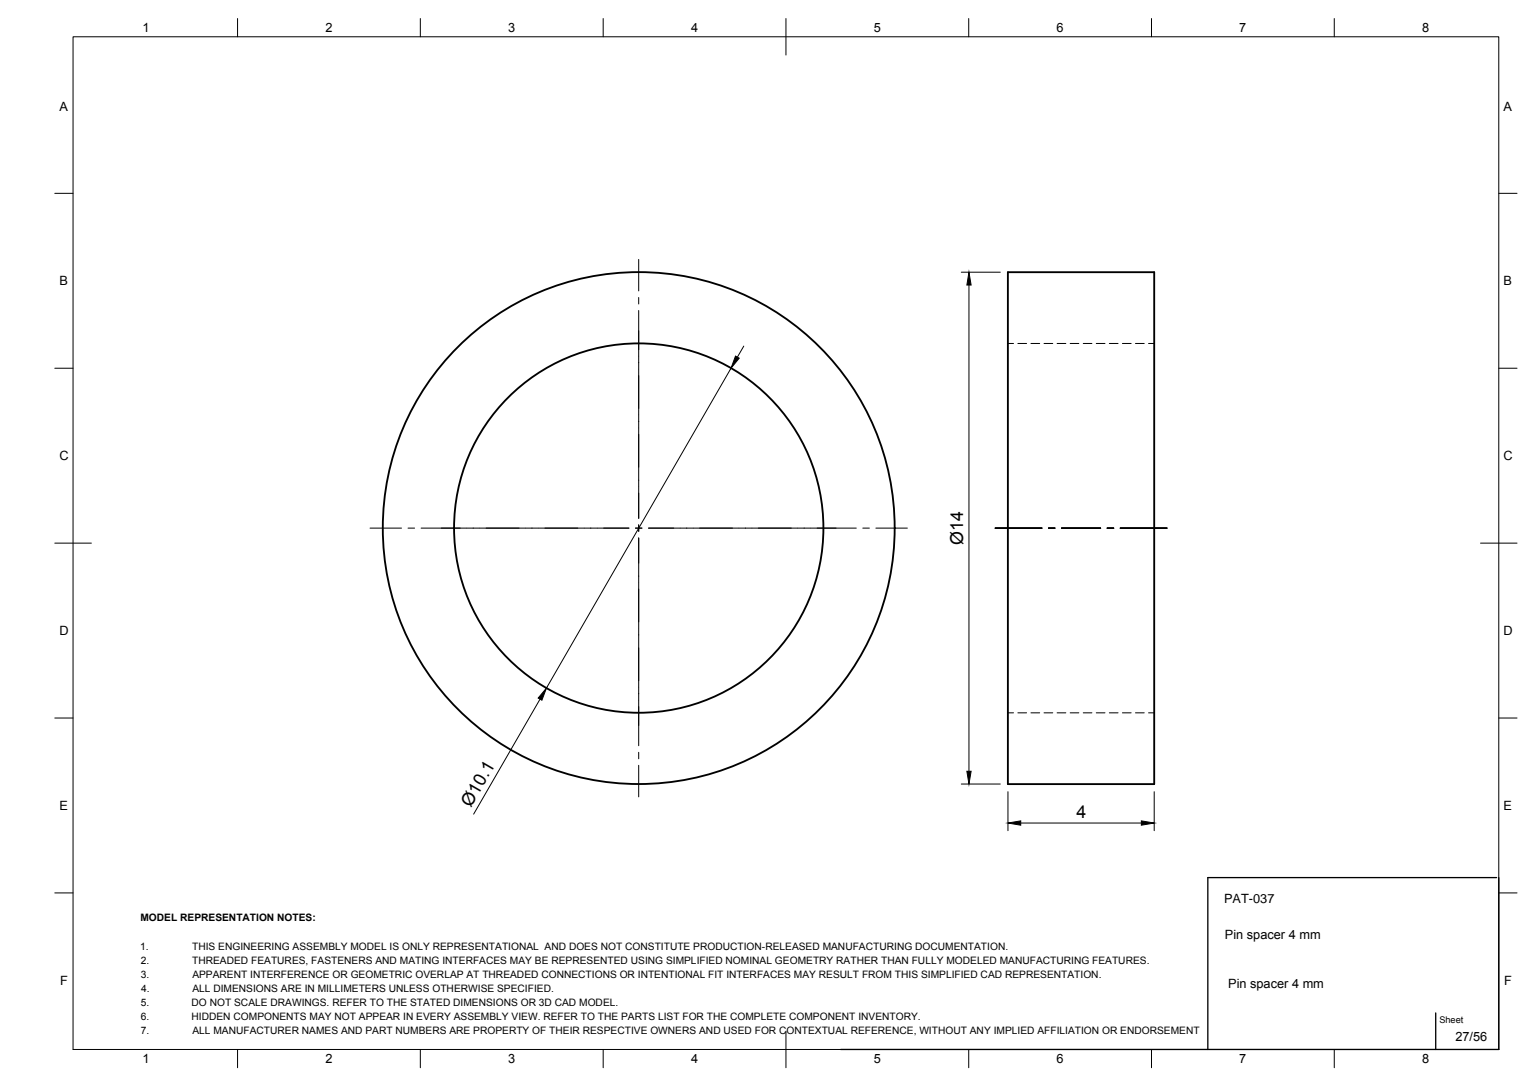
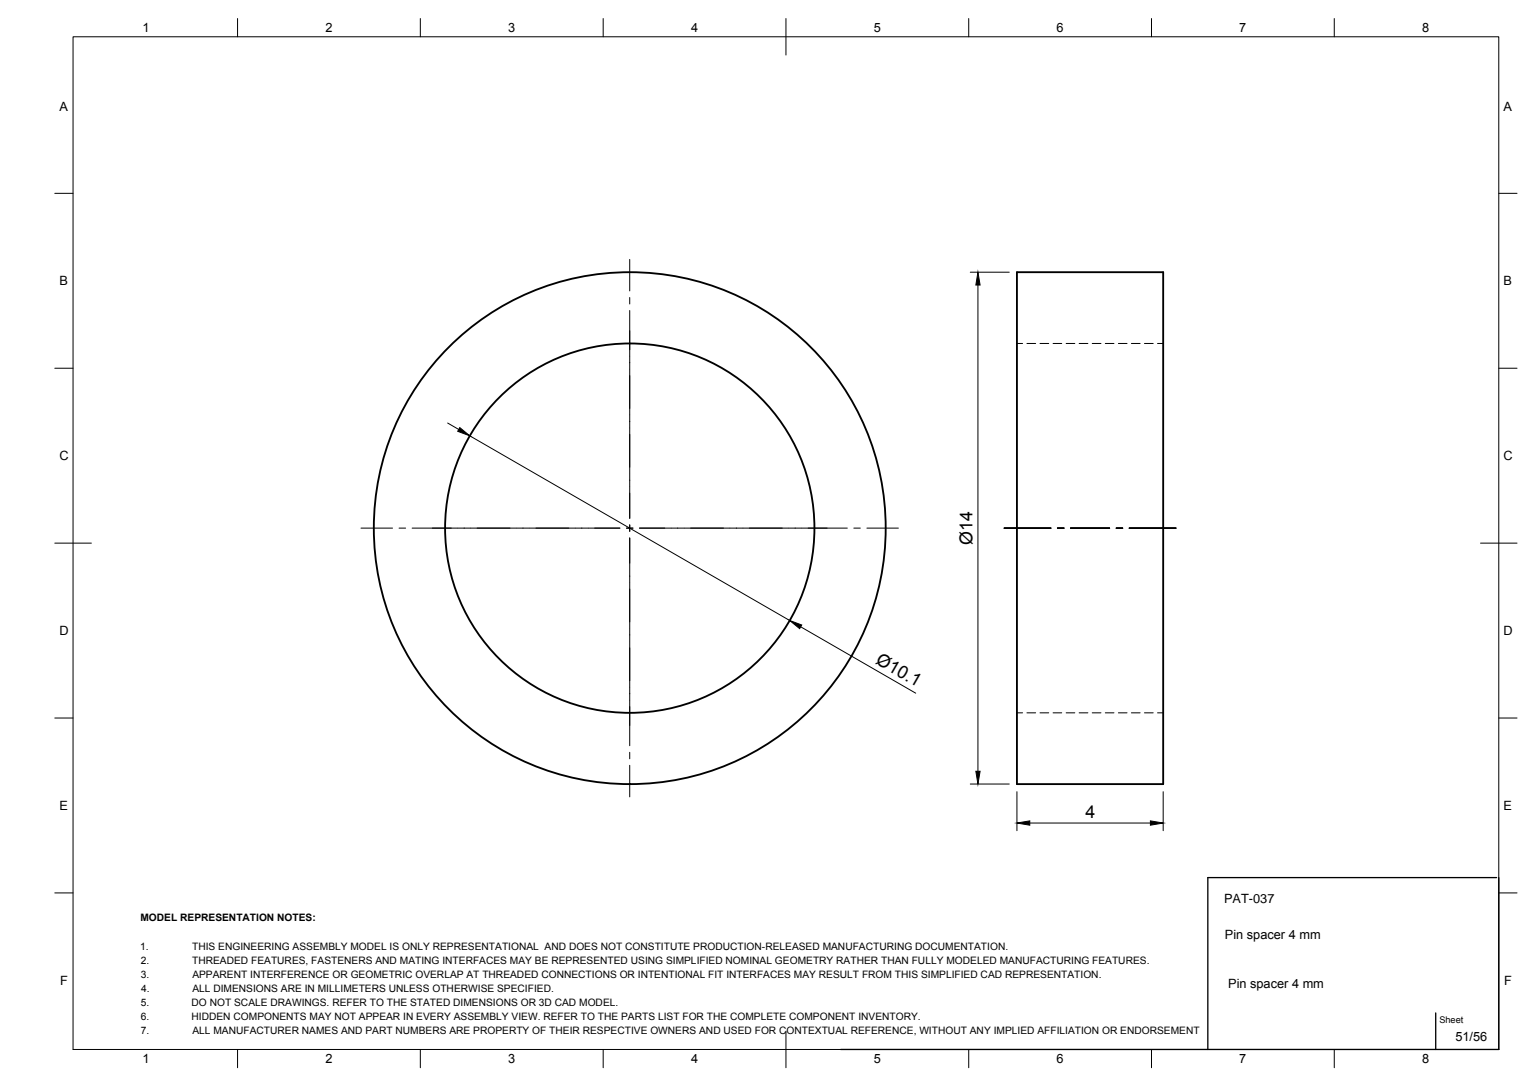
ISO-10303-21;
HEADER;
/* Generated by software containing ST-Developer
 * from STEP Tools, Inc. (www.steptools.com) 
 */

FILE_DESCRIPTION(
/* description */ ('Flywheel Crank-Slider'),
/* implementation_level */ '2;1');

FILE_NAME(
/* name */ 'Pin spacer 4 mm.step',
/* time_stamp */ '2026-10-28T03:23:13-07:00',
/* author */ (''),
/* organization */ (''),
/* preprocessor_version */ 'ST-DEVELOPER v20.2',
/* originating_system */ 'Autodesk Translation Framework v15.17.0.0',
/* authorisation */ '');

FILE_SCHEMA (('AUTOMOTIVE_DESIGN { 1 0 10303 214 3 1 1 }'));
ENDSEC;

DATA;
#10=MECHANICAL_DESIGN_GEOMETRIC_PRESENTATION_REPRESENTATION('',(#697),#17322);
#592=SHAPE_REPRESENTATION_RELATIONSHIP('SRR','None',#17590,#644);
#644=ADVANCED_BREP_SHAPE_REPRESENTATION('',(#754),#17294);
#697=STYLED_ITEM('',(#17931),#754);
#754=MANIFOLD_SOLID_BREP('Body1',#9079);
#926=FACE_BOUND('',#2327,.T.);
#927=FACE_BOUND('',#2329,.T.);
#1207=PLANE('',#10300);
#1208=PLANE('',#10301);
#1648=FACE_OUTER_BOUND('',#2324,.T.);
#1649=FACE_OUTER_BOUND('',#2325,.T.);
#1650=FACE_OUTER_BOUND('',#2326,.T.);
#1651=FACE_OUTER_BOUND('',#2328,.T.);
#2324=EDGE_LOOP('',(#7492,#7493,#7494,#7495));
#2325=EDGE_LOOP('',(#7496,#7497,#7498,#7499));
#2326=EDGE_LOOP('',(#7500));
#2327=EDGE_LOOP('',(#7501));
#2328=EDGE_LOOP('',(#7502));
#2329=EDGE_LOOP('',(#7503));
#3019=LINE('',#15818,#3630);
#3020=LINE('',#15824,#3631);
#3630=VECTOR('',#12455,0.505);
#3631=VECTOR('',#12462,0.7);
#4084=CIRCLE('',#10295,0.505);
#4085=CIRCLE('',#10296,0.505);
#4086=CIRCLE('',#10298,0.7);
#4087=CIRCLE('',#10299,0.7);
#4731=VERTEX_POINT('',#15815);
#4732=VERTEX_POINT('',#15817);
#4733=VERTEX_POINT('',#15821);
#4734=VERTEX_POINT('',#15823);
#5703=EDGE_CURVE('',#4731,#4731,#4084,.T.);
#5704=EDGE_CURVE('',#4731,#4732,#3019,.T.);
#5705=EDGE_CURVE('',#4732,#4732,#4085,.T.);
#5706=EDGE_CURVE('',#4733,#4733,#4086,.T.);
#5707=EDGE_CURVE('',#4733,#4734,#3020,.T.);
#5708=EDGE_CURVE('',#4734,#4734,#4087,.T.);
#7492=ORIENTED_EDGE('',*,*,#5703,.F.);
#7493=ORIENTED_EDGE('',*,*,#5704,.T.);
#7494=ORIENTED_EDGE('',*,*,#5705,.T.);
#7495=ORIENTED_EDGE('',*,*,#5704,.F.);
#7496=ORIENTED_EDGE('',*,*,#5706,.F.);
#7497=ORIENTED_EDGE('',*,*,#5707,.T.);
#7498=ORIENTED_EDGE('',*,*,#5708,.T.);
#7499=ORIENTED_EDGE('',*,*,#5707,.F.);
#7500=ORIENTED_EDGE('',*,*,#5706,.T.);
#7501=ORIENTED_EDGE('',*,*,#5703,.T.);
#7502=ORIENTED_EDGE('',*,*,#5708,.F.);
#7503=ORIENTED_EDGE('',*,*,#5705,.F.);
#8444=CYLINDRICAL_SURFACE('',#10294,0.505);
#8445=CYLINDRICAL_SURFACE('',#10297,0.7);
#8839=ADVANCED_FACE('',(#1648),#8444,.F.);
#8840=ADVANCED_FACE('',(#1649),#8445,.T.);
#8841=ADVANCED_FACE('',(#1650,#926),#1207,.T.);
#8842=ADVANCED_FACE('',(#1651,#927),#1208,.F.);
#9079=CLOSED_SHELL('',(#8839,#8840,#8841,#8842));
#10293=AXIS2_PLACEMENT_3D('',#15813,#12449,#12450);
#10294=AXIS2_PLACEMENT_3D('',#15814,#12451,#12452);
#10295=AXIS2_PLACEMENT_3D('',#15816,#12453,#12454);
#10296=AXIS2_PLACEMENT_3D('',#15819,#12456,#12457);
#10297=AXIS2_PLACEMENT_3D('',#15820,#12458,#12459);
#10298=AXIS2_PLACEMENT_3D('',#15822,#12460,#12461);
#10299=AXIS2_PLACEMENT_3D('',#15825,#12463,#12464);
#10300=AXIS2_PLACEMENT_3D('',#15826,#12465,#12466);
#10301=AXIS2_PLACEMENT_3D('',#15827,#12467,#12468);
#12449=DIRECTION('axis',(0.,0.,1.));
#12450=DIRECTION('refdir',(1.,0.,0.));
#12451=DIRECTION('center_axis',(0.,1.,0.));
#12452=DIRECTION('ref_axis',(1.,0.,0.));
#12453=DIRECTION('center_axis',(0.,-1.,0.));
#12454=DIRECTION('ref_axis',(1.,0.,0.));
#12455=DIRECTION('',(0.,-1.,0.));
#12456=DIRECTION('center_axis',(0.,-1.,0.));
#12457=DIRECTION('ref_axis',(1.,0.,0.));
#12458=DIRECTION('center_axis',(0.,1.,0.));
#12459=DIRECTION('ref_axis',(1.,0.,0.));
#12460=DIRECTION('center_axis',(0.,1.,0.));
#12461=DIRECTION('ref_axis',(1.,0.,0.));
#12462=DIRECTION('',(0.,-1.,0.));
#12463=DIRECTION('center_axis',(0.,1.,0.));
#12464=DIRECTION('ref_axis',(1.,0.,0.));
#12465=DIRECTION('center_axis',(0.,1.,0.));
#12466=DIRECTION('ref_axis',(1.,0.,0.));
#12467=DIRECTION('center_axis',(0.,1.,0.));
#12468=DIRECTION('ref_axis',(1.,0.,0.));
#15813=CARTESIAN_POINT('',(0.,0.,0.));
#15814=CARTESIAN_POINT('Origin',(2.,3.4,10.));
#15815=CARTESIAN_POINT('',(1.495,3.8,10.));
#15816=CARTESIAN_POINT('Origin',(2.,3.8,10.));
#15817=CARTESIAN_POINT('',(1.495,3.4,10.));
#15818=CARTESIAN_POINT('',(1.495,3.4,10.));
#15819=CARTESIAN_POINT('Origin',(2.,3.4,10.));
#15820=CARTESIAN_POINT('Origin',(2.,3.4,10.));
#15821=CARTESIAN_POINT('',(1.3,3.8,10.));
#15822=CARTESIAN_POINT('Origin',(2.,3.8,10.));
#15823=CARTESIAN_POINT('',(1.3,3.4,10.));
#15824=CARTESIAN_POINT('',(1.3,3.4,10.));
#15825=CARTESIAN_POINT('Origin',(2.,3.4,10.));
#15826=CARTESIAN_POINT('Origin',(2.,3.8,10.));
#15827=CARTESIAN_POINT('Origin',(2.,3.4,10.));
#17233=UNCERTAINTY_MEASURE_WITH_UNIT(LENGTH_MEASURE(0.001),#17323,
'DISTANCE_ACCURACY_VALUE',
'Maximum model space distance between geometric entities at asserted c
onnectivities');
#17261=UNCERTAINTY_MEASURE_WITH_UNIT(LENGTH_MEASURE(0.001),#17323,
'DISTANCE_ACCURACY_VALUE',
'Maximum model space distance between geometric entities at asserted c
onnectivities');
#17294=(
GEOMETRIC_REPRESENTATION_CONTEXT(3)
GLOBAL_UNCERTAINTY_ASSIGNED_CONTEXT((#17233))
GLOBAL_UNIT_ASSIGNED_CONTEXT((#17323,#17325,#17326))
REPRESENTATION_CONTEXT('','3D')
);
#17322=(
GEOMETRIC_REPRESENTATION_CONTEXT(3)
GLOBAL_UNCERTAINTY_ASSIGNED_CONTEXT((#17261))
GLOBAL_UNIT_ASSIGNED_CONTEXT((#17323,#17325,#17326))
REPRESENTATION_CONTEXT('','3D')
);
#17323=(
LENGTH_UNIT()
NAMED_UNIT(*)
SI_UNIT(.CENTI.,.METRE.)
);
#17325=(
NAMED_UNIT(*)
PLANE_ANGLE_UNIT()
SI_UNIT($,.RADIAN.)
);
#17326=(
NAMED_UNIT(*)
SI_UNIT($,.STERADIAN.)
SOLID_ANGLE_UNIT()
);
#17359=SHAPE_DEFINITION_REPRESENTATION(#17421,#17590);
#17421=PRODUCT_DEFINITION_SHAPE('',$,#17651);
#17590=SHAPE_REPRESENTATION('',(#10293),#17294);
#17618=PRODUCT_DEFINITION_CONTEXT('part definition',#17800,'design');
#17651=PRODUCT_DEFINITION('Pin spacer 4 mm','Pin spacer 4 mm',#17711,#17618);
#17711=PRODUCT_DEFINITION_FORMATION('',$,#17834);
#17800=APPLICATION_CONTEXT(
'Core Data for Automotive Mechanical Design Process');
#17801=PRODUCT_CONTEXT('part definition',#17800,'mechanical');
#17834=PRODUCT('Pin spacer 4 mm','Pin spacer 4 mm','Pin spacer 4 mm',(#17801));
#17925=COLOUR_RGB('Grey',0.48,0.52,0.57);
#17926=FILL_AREA_STYLE_COLOUR('',#17925);
#17927=FILL_AREA_STYLE('',(#17926));
#17928=SURFACE_STYLE_FILL_AREA(#17927);
#17929=SURFACE_SIDE_STYLE('',(#17928));
#17930=SURFACE_STYLE_USAGE(.BOTH.,#17929);
#17931=PRESENTATION_STYLE_ASSIGNMENT((#17930));
ENDSEC;
END-ISO-10303-21;
